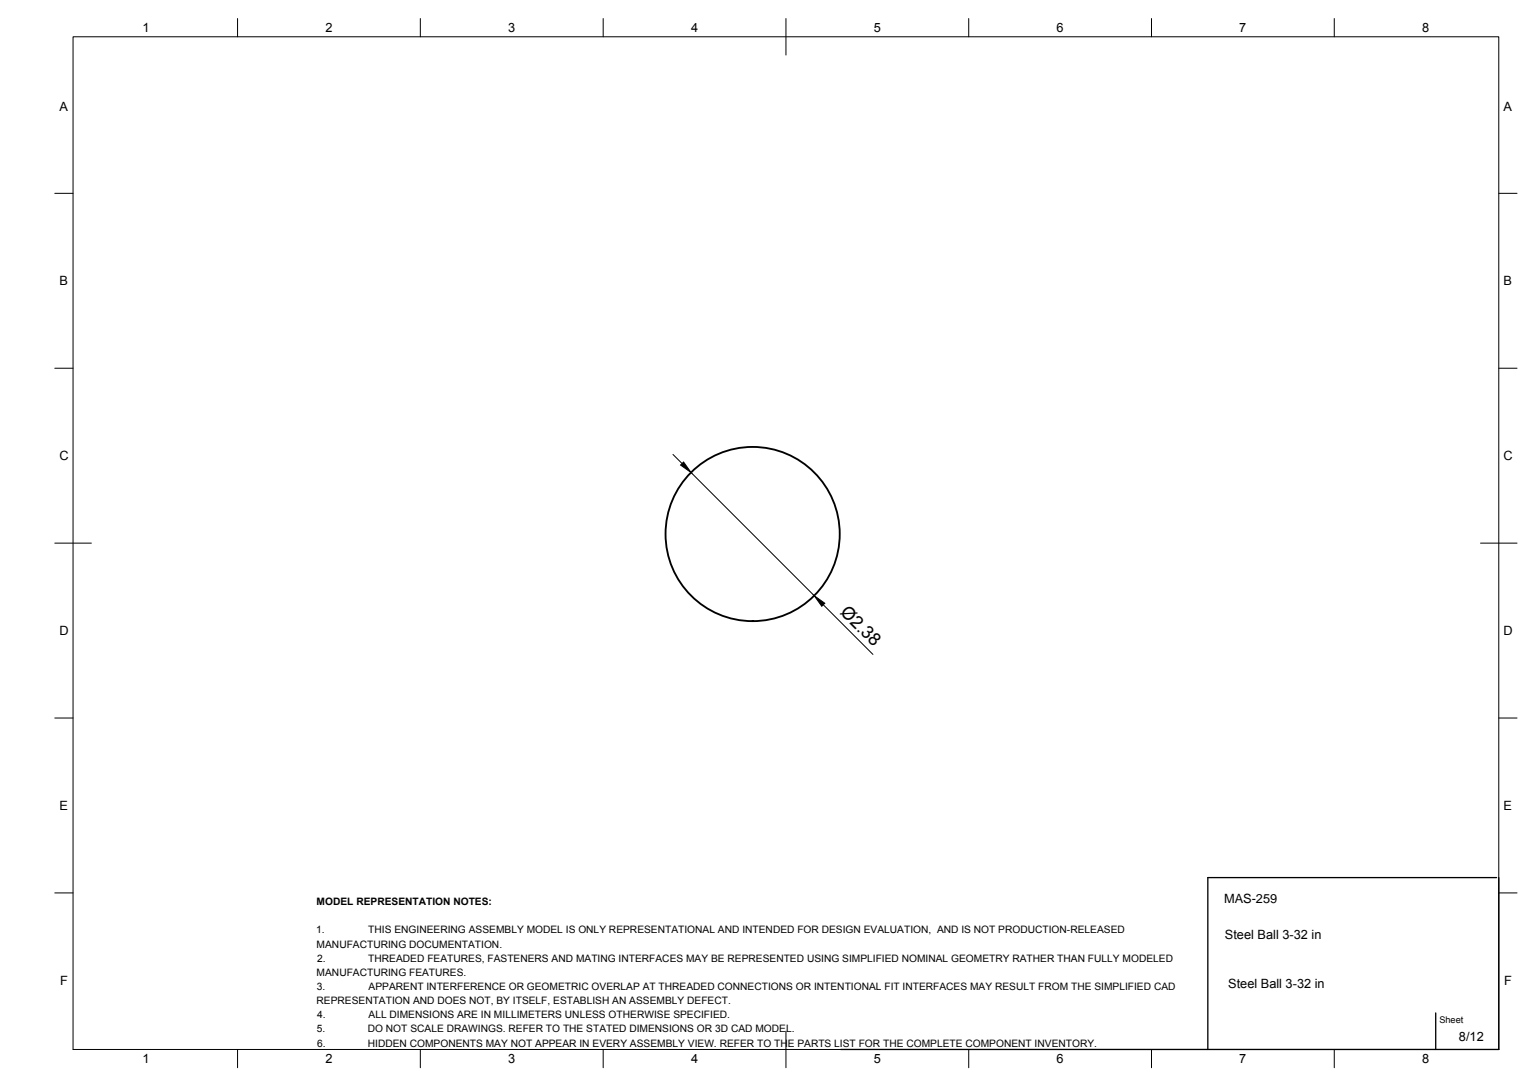
ISO-10303-21;
HEADER;
/* Generated by software containing ST-Developer
 * from STEP Tools, Inc. (www.steptools.com) 
 */

FILE_DESCRIPTION(
/* description */ (''),
/* implementation_level */ '2;1');

FILE_NAME(
/* name */ 'Steel Ball 3-32 in.step',
/* time_stamp */ '2026-10-15T13:30:17-07:00',
/* author */ (''),
/* organization */ (''),
/* preprocessor_version */ 'ST-DEVELOPER v20.2',
/* originating_system */ 'Autodesk Translation Framework v15.15.0.0',
/* authorisation */ '');

FILE_SCHEMA (('AUTOMOTIVE_DESIGN { 1 0 10303 214 3 1 1 }'));
ENDSEC;

DATA;
#10=MECHANICAL_DESIGN_GEOMETRIC_PRESENTATION_REPRESENTATION('',(#1039),#71795);
#1012=SPHERICAL_SURFACE('',#14112,1.190625);
#1019=SHAPE_REPRESENTATION_RELATIONSHIP('SRR','None',#72023,#1029);
#1029=ADVANCED_BREP_SHAPE_REPRESENTATION('',(#1049),#71791);
#1039=STYLED_ITEM('',(#72082),#1049);
#1049=MANIFOLD_SOLID_BREP('Body1',#13641);
#2212=FACE_OUTER_BOUND('',#2935,.T.);
#2935=EDGE_LOOP('',(#9857,#9858));
#3561=CIRCLE('',#14113,1.190625);
#5964=VERTEX_POINT('',#19888);
#5965=VERTEX_POINT('',#19889);
#7463=EDGE_CURVE('',#5964,#5965,#3561,.T.);
#9857=ORIENTED_EDGE('',*,*,#7463,.T.);
#9858=ORIENTED_EDGE('',*,*,#7463,.F.);
#13172=ADVANCED_FACE('',(#2212),#1012,.T.);
#13641=CLOSED_SHELL('',(#13172));
#14111=AXIS2_PLACEMENT_3D('',#19886,#15998,#15999);
#14112=AXIS2_PLACEMENT_3D('',#19887,#16000,#16001);
#14113=AXIS2_PLACEMENT_3D('',#19890,#16002,#16003);
#15998=DIRECTION('axis',(0.,0.,1.));
#15999=DIRECTION('refdir',(1.,0.,0.));
#16000=DIRECTION('center_axis',(0.,0.,1.));
#16001=DIRECTION('ref_axis',(1.,0.,0.));
#16002=DIRECTION('center_axis',(0.,-1.,0.));
#16003=DIRECTION('ref_axis',(-1.,0.,0.));
#19886=CARTESIAN_POINT('',(0.,0.,0.));
#19887=CARTESIAN_POINT('Origin',(42.8,14.9316563078761,40.0542456));
#19888=CARTESIAN_POINT('',(42.8,14.9316563078761,41.2448706));
#19889=CARTESIAN_POINT('',(42.8,14.9316563078761,38.8636206));
#19890=CARTESIAN_POINT('Origin',(42.8,14.9316563078761,40.0542456));
#71779=UNCERTAINTY_MEASURE_WITH_UNIT(LENGTH_MEASURE(0.01),#71796,
'DISTANCE_ACCURACY_VALUE',
'Maximum model space distance between geometric entities at asserted c
onnectivities');
#71783=UNCERTAINTY_MEASURE_WITH_UNIT(LENGTH_MEASURE(0.01),#71796,
'DISTANCE_ACCURACY_VALUE',
'Maximum model space distance between geometric entities at asserted c
onnectivities');
#71791=(
GEOMETRIC_REPRESENTATION_CONTEXT(3)
GLOBAL_UNCERTAINTY_ASSIGNED_CONTEXT((#71779))
GLOBAL_UNIT_ASSIGNED_CONTEXT((#71796,#71798,#71799))
REPRESENTATION_CONTEXT('','3D')
);
#71795=(
GEOMETRIC_REPRESENTATION_CONTEXT(3)
GLOBAL_UNCERTAINTY_ASSIGNED_CONTEXT((#71783))
GLOBAL_UNIT_ASSIGNED_CONTEXT((#71796,#71798,#71799))
REPRESENTATION_CONTEXT('','3D')
);
#71796=(
LENGTH_UNIT()
NAMED_UNIT(*)
SI_UNIT(.MILLI.,.METRE.)
);
#71798=(
NAMED_UNIT(*)
PLANE_ANGLE_UNIT()
SI_UNIT($,.RADIAN.)
);
#71799=(
NAMED_UNIT(*)
SI_UNIT($,.STERADIAN.)
SOLID_ANGLE_UNIT()
);
#71807=SHAPE_DEFINITION_REPRESENTATION(#71818,#72023);
#71818=PRODUCT_DEFINITION_SHAPE('',$,#72035);
#72023=SHAPE_REPRESENTATION('',(#14111),#71791);
#72027=PRODUCT_DEFINITION_CONTEXT('part definition',#72062,'design');
#72035=PRODUCT_DEFINITION('Steel Ball 3-32 in','Steel Ball 3-32 in',#72046,
#72027);
#72046=PRODUCT_DEFINITION_FORMATION('',$,#72071);
#72062=APPLICATION_CONTEXT(
'Core Data for Automotive Mechanical Design Process');
#72063=PRODUCT_CONTEXT('part definition',#72062,'mechanical');
#72071=PRODUCT('Steel Ball 3-32 in','Steel Ball 3-32 in',$,(#72063));
#72082=PRESENTATION_STYLE_ASSIGNMENT((#72093));
#72093=SURFACE_STYLE_USAGE(.BOTH.,#72104);
#72104=SURFACE_SIDE_STYLE('',(#72115));
#72115=SURFACE_STYLE_FILL_AREA(#72126);
#72126=FILL_AREA_STYLE('Opaque(240,241,243)',(#72137));
#72137=FILL_AREA_STYLE_COLOUR('Opaque(240,241,243)',#72148);
#72148=COLOUR_RGB('Opaque(240,241,243)', 0.09019608, 0.27058824, 0.51372549);
ENDSEC;
END-ISO-10303-21;
